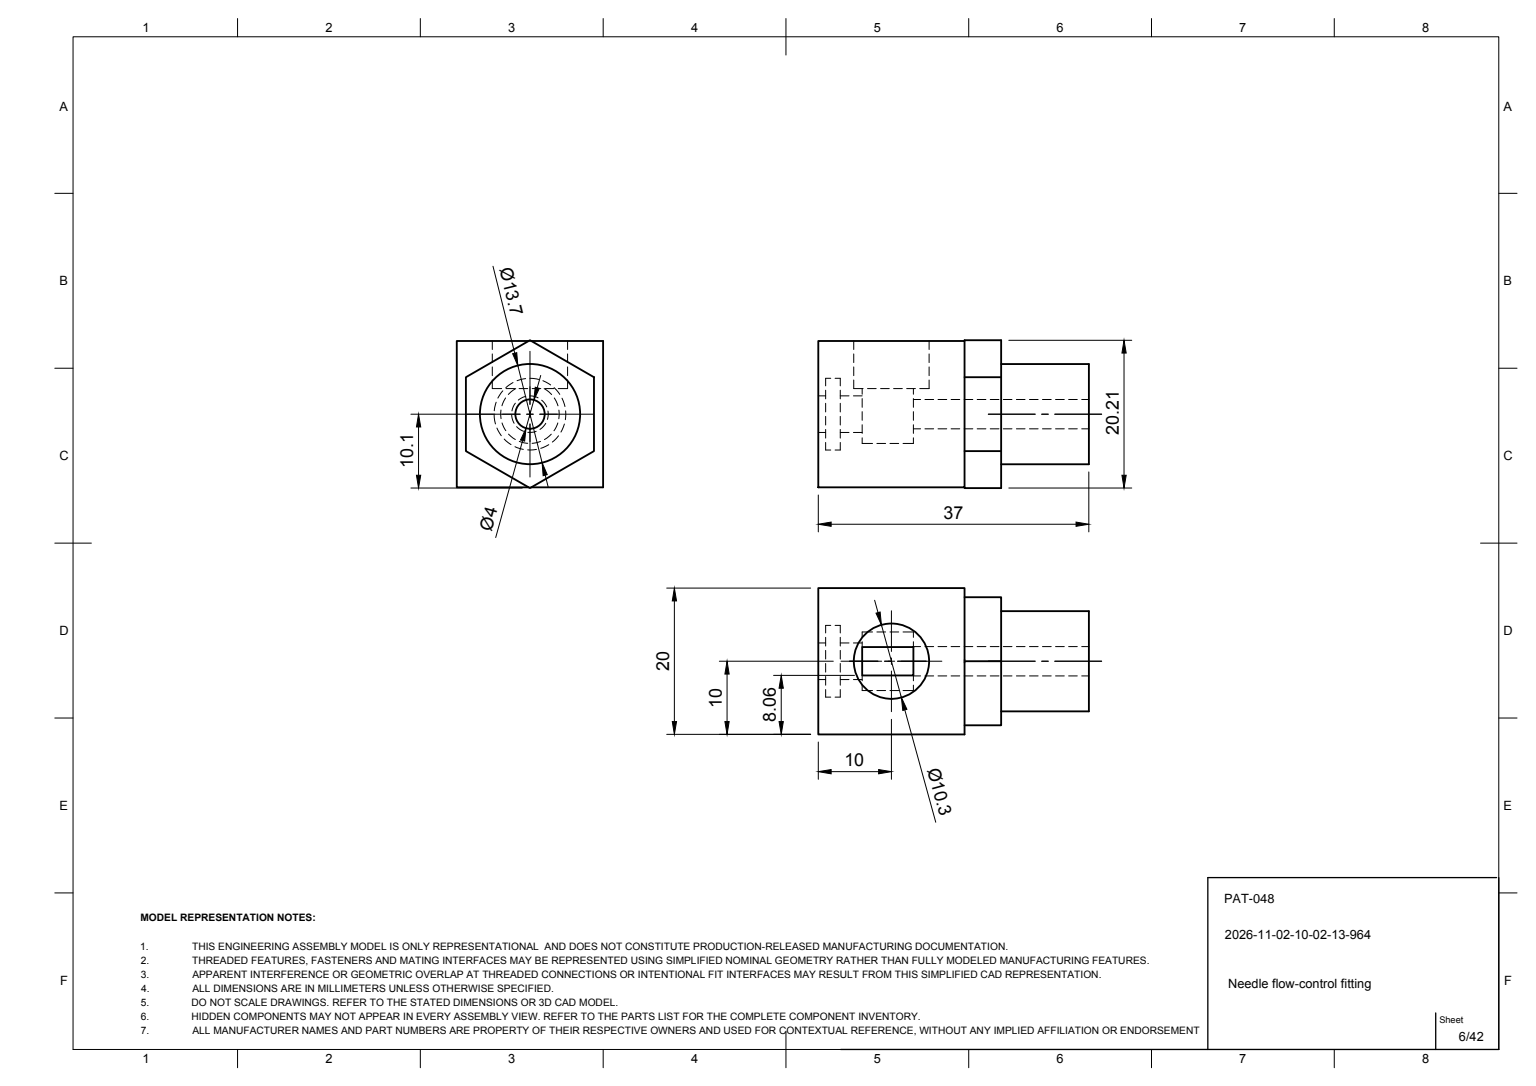
ISO-10303-21;
HEADER;
/* Generated by software containing ST-Developer
 * from STEP Tools, Inc. (www.steptools.com) 
 */

FILE_DESCRIPTION(
/* description */ ('Guided pneumatic stop gate'),
/* implementation_level */ '2;1');

FILE_NAME(
/* name */ 'Needle flow-control fitting.step',
/* time_stamp */ '2026-10-27T21:43:45-07:00',
/* author */ (''),
/* organization */ (''),
/* preprocessor_version */ 'ST-DEVELOPER v20.2',
/* originating_system */ 'Autodesk Translation Framework v15.17.0.0',
/* authorisation */ '');

FILE_SCHEMA (('AUTOMOTIVE_DESIGN { 1 0 10303 214 3 1 1 }'));
ENDSEC;

DATA;
#10=MECHANICAL_DESIGN_GEOMETRIC_PRESENTATION_REPRESENTATION('',(#536),#14392);
#452=SHAPE_REPRESENTATION_RELATIONSHIP('SRR','None',#14586,#494);
#494=ADVANCED_BREP_SHAPE_REPRESENTATION('',(#578),#14348);
#536=STYLED_ITEM('',(#14884),#578);
#578=MANIFOLD_SOLID_BREP('Body1',#7876);
#630=FACE_BOUND('',#1642,.T.);
#631=FACE_BOUND('',#1644,.T.);
#632=FACE_BOUND('',#1648,.T.);
#633=FACE_BOUND('',#1650,.T.);
#634=FACE_BOUND('',#1654,.T.);
#635=FACE_BOUND('',#1658,.T.);
#636=FACE_BOUND('',#1662,.T.);
#637=FACE_BOUND('',#1666,.T.);
#638=FACE_BOUND('',#1677,.T.);
#856=PLANE('',#8460);
#857=PLANE('',#8461);
#858=PLANE('',#8469);
#859=PLANE('',#8471);
#860=PLANE('',#8476);
#861=PLANE('',#8478);
#862=PLANE('',#8479);
#863=PLANE('',#8480);
#864=PLANE('',#8481);
#865=PLANE('',#8482);
#866=PLANE('',#8483);
#867=PLANE('',#8484);
#868=PLANE('',#8485);
#869=PLANE('',#8486);
#870=PLANE('',#8488);
#871=PLANE('',#8489);
#872=PLANE('',#8490);
#873=PLANE('',#8491);
#874=PLANE('',#8492);
#875=PLANE('',#8493);
#876=PLANE('',#8494);
#877=PLANE('',#8499);
#1150=FACE_OUTER_BOUND('',#1640,.T.);
#1151=FACE_OUTER_BOUND('',#1641,.T.);
#1152=FACE_OUTER_BOUND('',#1643,.T.);
#1153=FACE_OUTER_BOUND('',#1645,.T.);
#1154=FACE_OUTER_BOUND('',#1646,.T.);
#1155=FACE_OUTER_BOUND('',#1647,.T.);
#1156=FACE_OUTER_BOUND('',#1649,.T.);
#1157=FACE_OUTER_BOUND('',#1651,.T.);
#1158=FACE_OUTER_BOUND('',#1652,.T.);
#1159=FACE_OUTER_BOUND('',#1653,.T.);
#1160=FACE_OUTER_BOUND('',#1655,.T.);
#1161=FACE_OUTER_BOUND('',#1656,.T.);
#1162=FACE_OUTER_BOUND('',#1657,.T.);
#1163=FACE_OUTER_BOUND('',#1659,.T.);
#1164=FACE_OUTER_BOUND('',#1660,.T.);
#1165=FACE_OUTER_BOUND('',#1661,.T.);
#1166=FACE_OUTER_BOUND('',#1663,.T.);
#1167=FACE_OUTER_BOUND('',#1664,.T.);
#1168=FACE_OUTER_BOUND('',#1665,.T.);
#1169=FACE_OUTER_BOUND('',#1667,.T.);
#1170=FACE_OUTER_BOUND('',#1668,.T.);
#1171=FACE_OUTER_BOUND('',#1669,.T.);
#1172=FACE_OUTER_BOUND('',#1670,.T.);
#1173=FACE_OUTER_BOUND('',#1671,.T.);
#1174=FACE_OUTER_BOUND('',#1672,.T.);
#1175=FACE_OUTER_BOUND('',#1673,.T.);
#1176=FACE_OUTER_BOUND('',#1674,.T.);
#1177=FACE_OUTER_BOUND('',#1675,.T.);
#1178=FACE_OUTER_BOUND('',#1676,.T.);
#1640=EDGE_LOOP('',(#5450,#5451,#5452,#5453));
#1641=EDGE_LOOP('',(#5454));
#1642=EDGE_LOOP('',(#5455,#5456,#5457,#5458));
#1643=EDGE_LOOP('',(#5459,#5460));
#1644=EDGE_LOOP('',(#5461));
#1645=EDGE_LOOP('',(#5462,#5463,#5464,#5465));
#1646=EDGE_LOOP('',(#5466,#5467,#5468,#5469));
#1647=EDGE_LOOP('',(#5470));
#1648=EDGE_LOOP('',(#5471));
#1649=EDGE_LOOP('',(#5472));
#1650=EDGE_LOOP('',(#5473));
#1651=EDGE_LOOP('',(#5474,#5475,#5476,#5477));
#1652=EDGE_LOOP('',(#5478,#5479,#5480,#5481));
#1653=EDGE_LOOP('',(#5482,#5483));
#1654=EDGE_LOOP('',(#5484));
#1655=EDGE_LOOP('',(#5485,#5486,#5487,#5488,#5489,#5490));
#1656=EDGE_LOOP('',(#5491,#5492,#5493,#5494));
#1657=EDGE_LOOP('',(#5495,#5496,#5497,#5498,#5499,#5500));
#1658=EDGE_LOOP('',(#5501));
#1659=EDGE_LOOP('',(#5502,#5503,#5504,#5505));
#1660=EDGE_LOOP('',(#5506,#5507,#5508,#5509,#5510,#5511));
#1661=EDGE_LOOP('',(#5512,#5513,#5514,#5515));
#1662=EDGE_LOOP('',(#5516));
#1663=EDGE_LOOP('',(#5517,#5518,#5519,#5520,#5521,#5522));
#1664=EDGE_LOOP('',(#5523,#5524,#5525));
#1665=EDGE_LOOP('',(#5526,#5527,#5528,#5529,#5530,#5531));
#1666=EDGE_LOOP('',(#5532));
#1667=EDGE_LOOP('',(#5533,#5534,#5535,#5536));
#1668=EDGE_LOOP('',(#5537,#5538,#5539,#5540,#5541));
#1669=EDGE_LOOP('',(#5542,#5543,#5544,#5545,#5546));
#1670=EDGE_LOOP('',(#5547,#5548,#5549,#5550));
#1671=EDGE_LOOP('',(#5551,#5552,#5553,#5554,#5555));
#1672=EDGE_LOOP('',(#5556,#5557,#5558,#5559,#5560));
#1673=EDGE_LOOP('',(#5561,#5562,#5563));
#1674=EDGE_LOOP('',(#5564,#5565,#5566,#5567));
#1675=EDGE_LOOP('',(#5568,#5569,#5570,#5571));
#1676=EDGE_LOOP('',(#5572));
#1677=EDGE_LOOP('',(#5573));
#2308=LINE('',#12067,#2853);
#2309=LINE('',#12072,#2854);
#2310=LINE('',#12074,#2855);
#2311=LINE('',#12076,#2856);
#2312=LINE('',#12077,#2857);
#2313=LINE('',#12088,#2858);
#2314=LINE('',#12097,#2859);
#2315=LINE('',#12100,#2860);
#2316=LINE('',#12108,#2861);
#2317=LINE('',#12110,#2862);
#2318=LINE('',#12112,#2863);
#2319=LINE('',#12114,#2864);
#2320=LINE('',#12116,#2865);
#2321=LINE('',#12117,#2866);
#2322=LINE('',#12121,#2867);
#2323=LINE('',#12123,#2868);
#2324=LINE('',#12125,#2869);
#2325=LINE('',#12126,#2870);
#2326=LINE('',#12129,#2871);
#2327=LINE('',#12130,#2872);
#2328=LINE('',#12132,#2873);
#2329=LINE('',#12133,#2874);
#2330=LINE('',#12136,#2875);
#2331=LINE('',#12137,#2876);
#2332=LINE('',#12140,#2877);
#2333=LINE('',#12141,#2878);
#2334=LINE('',#12142,#2879);
#2335=LINE('',#12146,#2880);
#2336=LINE('',#12148,#2881);
#2337=LINE('',#12149,#2882);
#2338=LINE('',#12152,#2883);
#2339=LINE('',#12153,#2884);
#2340=LINE('',#12157,#2885);
#2341=LINE('',#12159,#2886);
#2342=LINE('',#12161,#2887);
#2343=LINE('',#12163,#2888);
#2344=LINE('',#12165,#2889);
#2345=LINE('',#12166,#2890);
#2346=LINE('',#12170,#2891);
#2347=LINE('',#12171,#2892);
#2348=LINE('',#12174,#2893);
#2349=LINE('',#12175,#2894);
#2350=LINE('',#12177,#2895);
#2351=LINE('',#12178,#2896);
#2352=LINE('',#12180,#2897);
#2353=LINE('',#12182,#2898);
#2354=LINE('',#12187,#2899);
#2355=LINE('',#12191,#2900);
#2853=VECTOR('',#9561,0.515);
#2854=VECTOR('',#9566,1.);
#2855=VECTOR('',#9567,1.);
#2856=VECTOR('',#9568,1.);
#2857=VECTOR('',#9569,1.);
#2858=VECTOR('',#9584,0.49);
#2859=VECTOR('',#9597,0.25);
#2860=VECTOR('',#9600,0.25);
#2861=VECTOR('',#9609,1.);
#2862=VECTOR('',#9610,1.);
#2863=VECTOR('',#9611,1.);
#2864=VECTOR('',#9612,1.);
#2865=VECTOR('',#9613,1.);
#2866=VECTOR('',#9614,1.);
#2867=VECTOR('',#9617,1.);
#2868=VECTOR('',#9618,1.);
#2869=VECTOR('',#9619,1.);
#2870=VECTOR('',#9620,1.);
#2871=VECTOR('',#9623,1.);
#2872=VECTOR('',#9624,1.);
#2873=VECTOR('',#9625,1.);
#2874=VECTOR('',#9626,1.);
#2875=VECTOR('',#9629,1.);
#2876=VECTOR('',#9630,1.);
#2877=VECTOR('',#9633,1.);
#2878=VECTOR('',#9634,1.);
#2879=VECTOR('',#9635,1.);
#2880=VECTOR('',#9640,1.);
#2881=VECTOR('',#9641,1.);
#2882=VECTOR('',#9642,1.);
#2883=VECTOR('',#9645,1.);
#2884=VECTOR('',#9646,1.);
#2885=VECTOR('',#9649,1.);
#2886=VECTOR('',#9650,1.);
#2887=VECTOR('',#9651,1.);
#2888=VECTOR('',#9652,1.);
#2889=VECTOR('',#9653,1.);
#2890=VECTOR('',#9654,1.);
#2891=VECTOR('',#9659,1.);
#2892=VECTOR('',#9660,1.);
#2893=VECTOR('',#9663,1.);
#2894=VECTOR('',#9664,1.);
#2895=VECTOR('',#9667,1.);
#2896=VECTOR('',#9668,1.);
#2897=VECTOR('',#9671,1.);
#2898=VECTOR('',#9674,1.);
#2899=VECTOR('',#9681,0.2);
#2900=VECTOR('',#9686,0.685);
#3398=CIRCLE('',#8458,0.515);
#3399=CIRCLE('',#8459,0.515);
#3400=CIRCLE('',#8462,0.4);
#3401=CIRCLE('',#8463,0.25);
#3402=CIRCLE('',#8465,0.4);
#3403=CIRCLE('',#8467,0.49);
#3404=CIRCLE('',#8468,0.49);
#3405=CIRCLE('',#8470,0.25);
#3406=CIRCLE('',#8472,0.25);
#3407=CIRCLE('',#8475,0.25);
#3408=CIRCLE('',#8477,0.2);
#3409=CIRCLE('',#8487,0.685);
#3410=CIRCLE('',#8496,0.2);
#3411=CIRCLE('',#8498,0.685);
#3777=VERTEX_POINT('',#12064);
#3778=VERTEX_POINT('',#12066);
#3779=VERTEX_POINT('',#12070);
#3780=VERTEX_POINT('',#12071);
#3781=VERTEX_POINT('',#12073);
#3782=VERTEX_POINT('',#12075);
#3783=VERTEX_POINT('',#12080);
#3784=VERTEX_POINT('',#12085);
#3785=VERTEX_POINT('',#12087);
#3786=VERTEX_POINT('',#12091);
#3787=VERTEX_POINT('',#12094);
#3788=VERTEX_POINT('',#12099);
#3789=VERTEX_POINT('',#12103);
#3790=VERTEX_POINT('',#12106);
#3791=VERTEX_POINT('',#12107);
#3792=VERTEX_POINT('',#12109);
#3793=VERTEX_POINT('',#12111);
#3794=VERTEX_POINT('',#12113);
#3795=VERTEX_POINT('',#12115);
#3796=VERTEX_POINT('',#12119);
#3797=VERTEX_POINT('',#12120);
#3798=VERTEX_POINT('',#12122);
#3799=VERTEX_POINT('',#12124);
#3800=VERTEX_POINT('',#12128);
#3801=VERTEX_POINT('',#12131);
#3802=VERTEX_POINT('',#12135);
#3803=VERTEX_POINT('',#12139);
#3804=VERTEX_POINT('',#12145);
#3805=VERTEX_POINT('',#12147);
#3806=VERTEX_POINT('',#12151);
#3807=VERTEX_POINT('',#12155);
#3808=VERTEX_POINT('',#12156);
#3809=VERTEX_POINT('',#12158);
#3810=VERTEX_POINT('',#12160);
#3811=VERTEX_POINT('',#12162);
#3812=VERTEX_POINT('',#12164);
#3813=VERTEX_POINT('',#12167);
#3814=VERTEX_POINT('',#12173);
#3815=VERTEX_POINT('',#12186);
#3816=VERTEX_POINT('',#12190);
#4423=EDGE_CURVE('',#3777,#3777,#3398,.T.);
#4424=EDGE_CURVE('',#3777,#3778,#2308,.T.);
#4425=EDGE_CURVE('',#3778,#3778,#3399,.T.);
#4426=EDGE_CURVE('',#3779,#3780,#2309,.T.);
#4427=EDGE_CURVE('',#3781,#3779,#2310,.T.);
#4428=EDGE_CURVE('',#3782,#3781,#2311,.T.);
#4429=EDGE_CURVE('',#3780,#3782,#2312,.T.);
#4430=EDGE_CURVE('',#3781,#3779,#3400,.T.);
#4431=EDGE_CURVE('',#3783,#3783,#3401,.T.);
#4432=EDGE_CURVE('',#3782,#3780,#3402,.T.);
#4433=EDGE_CURVE('',#3784,#3784,#3403,.T.);
#4434=EDGE_CURVE('',#3784,#3785,#2313,.T.);
#4435=EDGE_CURVE('',#3785,#3785,#3404,.T.);
#4436=EDGE_CURVE('',#3786,#3786,#3405,.T.);
#4437=EDGE_CURVE('',#3787,#3787,#3406,.T.);
#4438=EDGE_CURVE('',#3783,#3787,#2314,.T.);
#4439=EDGE_CURVE('',#3786,#3788,#2315,.T.);
#4440=EDGE_CURVE('',#3788,#3788,#3407,.T.);
#4441=EDGE_CURVE('',#3789,#3789,#3408,.T.);
#4442=EDGE_CURVE('',#3790,#3791,#2316,.T.);
#4443=EDGE_CURVE('',#3791,#3792,#2317,.T.);
#4444=EDGE_CURVE('',#3792,#3793,#2318,.T.);
#4445=EDGE_CURVE('',#3794,#3793,#2319,.T.);
#4446=EDGE_CURVE('',#3795,#3794,#2320,.T.);
#4447=EDGE_CURVE('',#3790,#3795,#2321,.T.);
#4448=EDGE_CURVE('',#3796,#3797,#2322,.T.);
#4449=EDGE_CURVE('',#3797,#3798,#2323,.T.);
#4450=EDGE_CURVE('',#3799,#3798,#2324,.T.);
#4451=EDGE_CURVE('',#3796,#3799,#2325,.T.);
#4452=EDGE_CURVE('',#3800,#3793,#2326,.T.);
#4453=EDGE_CURVE('',#3800,#3796,#2327,.T.);
#4454=EDGE_CURVE('',#3801,#3799,#2328,.T.);
#4455=EDGE_CURVE('',#3794,#3801,#2329,.T.);
#4456=EDGE_CURVE('',#3802,#3801,#2330,.T.);
#4457=EDGE_CURVE('',#3795,#3802,#2331,.T.);
#4458=EDGE_CURVE('',#3797,#3803,#2332,.T.);
#4459=EDGE_CURVE('',#3790,#3803,#2333,.T.);
#4460=EDGE_CURVE('',#3798,#3802,#2334,.T.);
#4461=EDGE_CURVE('',#3804,#3803,#2335,.T.);
#4462=EDGE_CURVE('',#3800,#3805,#2336,.T.);
#4463=EDGE_CURVE('',#3805,#3804,#2337,.T.);
#4464=EDGE_CURVE('',#3793,#3806,#2338,.T.);
#4465=EDGE_CURVE('',#3806,#3800,#2339,.T.);
#4466=EDGE_CURVE('',#3807,#3808,#2340,.T.);
#4467=EDGE_CURVE('',#3809,#3807,#2341,.T.);
#4468=EDGE_CURVE('',#3810,#3809,#2342,.T.);
#4469=EDGE_CURVE('',#3811,#3810,#2343,.T.);
#4470=EDGE_CURVE('',#3812,#3811,#2344,.T.);
#4471=EDGE_CURVE('',#3808,#3812,#2345,.T.);
#4472=EDGE_CURVE('',#3813,#3813,#3409,.T.);
#4473=EDGE_CURVE('',#3807,#3792,#2346,.T.);
#4474=EDGE_CURVE('',#3809,#3791,#2347,.T.);
#4475=EDGE_CURVE('',#3814,#3790,#2348,.T.);
#4476=EDGE_CURVE('',#3810,#3814,#2349,.T.);
#4477=EDGE_CURVE('',#3803,#3814,#2350,.T.);
#4478=EDGE_CURVE('',#3811,#3804,#2351,.T.);
#4479=EDGE_CURVE('',#3812,#3805,#2352,.T.);
#4480=EDGE_CURVE('',#3808,#3806,#2353,.T.);
#4481=EDGE_CURVE('',#3789,#3815,#2354,.T.);
#4482=EDGE_CURVE('',#3815,#3815,#3410,.T.);
#4483=EDGE_CURVE('',#3813,#3816,#2355,.T.);
#4484=EDGE_CURVE('',#3816,#3816,#3411,.T.);
#5450=ORIENTED_EDGE('',*,*,#4423,.F.);
#5451=ORIENTED_EDGE('',*,*,#4424,.T.);
#5452=ORIENTED_EDGE('',*,*,#4425,.F.);
#5453=ORIENTED_EDGE('',*,*,#4424,.F.);
#5454=ORIENTED_EDGE('',*,*,#4423,.T.);
#5455=ORIENTED_EDGE('',*,*,#4426,.F.);
#5456=ORIENTED_EDGE('',*,*,#4427,.F.);
#5457=ORIENTED_EDGE('',*,*,#4428,.F.);
#5458=ORIENTED_EDGE('',*,*,#4429,.F.);
#5459=ORIENTED_EDGE('',*,*,#4427,.T.);
#5460=ORIENTED_EDGE('',*,*,#4430,.F.);
#5461=ORIENTED_EDGE('',*,*,#4431,.T.);
#5462=ORIENTED_EDGE('',*,*,#4428,.T.);
#5463=ORIENTED_EDGE('',*,*,#4430,.T.);
#5464=ORIENTED_EDGE('',*,*,#4426,.T.);
#5465=ORIENTED_EDGE('',*,*,#4432,.F.);
#5466=ORIENTED_EDGE('',*,*,#4433,.F.);
#5467=ORIENTED_EDGE('',*,*,#4434,.T.);
#5468=ORIENTED_EDGE('',*,*,#4435,.T.);
#5469=ORIENTED_EDGE('',*,*,#4434,.F.);
#5470=ORIENTED_EDGE('',*,*,#4435,.F.);
#5471=ORIENTED_EDGE('',*,*,#4436,.F.);
#5472=ORIENTED_EDGE('',*,*,#4433,.T.);
#5473=ORIENTED_EDGE('',*,*,#4437,.F.);
#5474=ORIENTED_EDGE('',*,*,#4431,.F.);
#5475=ORIENTED_EDGE('',*,*,#4438,.T.);
#5476=ORIENTED_EDGE('',*,*,#4437,.T.);
#5477=ORIENTED_EDGE('',*,*,#4438,.F.);
#5478=ORIENTED_EDGE('',*,*,#4436,.T.);
#5479=ORIENTED_EDGE('',*,*,#4439,.T.);
#5480=ORIENTED_EDGE('',*,*,#4440,.F.);
#5481=ORIENTED_EDGE('',*,*,#4439,.F.);
#5482=ORIENTED_EDGE('',*,*,#4429,.T.);
#5483=ORIENTED_EDGE('',*,*,#4432,.T.);
#5484=ORIENTED_EDGE('',*,*,#4441,.F.);
#5485=ORIENTED_EDGE('',*,*,#4442,.T.);
#5486=ORIENTED_EDGE('',*,*,#4443,.T.);
#5487=ORIENTED_EDGE('',*,*,#4444,.T.);
#5488=ORIENTED_EDGE('',*,*,#4445,.F.);
#5489=ORIENTED_EDGE('',*,*,#4446,.F.);
#5490=ORIENTED_EDGE('',*,*,#4447,.F.);
#5491=ORIENTED_EDGE('',*,*,#4448,.T.);
#5492=ORIENTED_EDGE('',*,*,#4449,.T.);
#5493=ORIENTED_EDGE('',*,*,#4450,.F.);
#5494=ORIENTED_EDGE('',*,*,#4451,.F.);
#5495=ORIENTED_EDGE('',*,*,#4445,.T.);
#5496=ORIENTED_EDGE('',*,*,#4452,.F.);
#5497=ORIENTED_EDGE('',*,*,#4453,.T.);
#5498=ORIENTED_EDGE('',*,*,#4451,.T.);
#5499=ORIENTED_EDGE('',*,*,#4454,.F.);
#5500=ORIENTED_EDGE('',*,*,#4455,.F.);
#5501=ORIENTED_EDGE('',*,*,#4425,.T.);
#5502=ORIENTED_EDGE('',*,*,#4446,.T.);
#5503=ORIENTED_EDGE('',*,*,#4455,.T.);
#5504=ORIENTED_EDGE('',*,*,#4456,.F.);
#5505=ORIENTED_EDGE('',*,*,#4457,.F.);
#5506=ORIENTED_EDGE('',*,*,#4458,.T.);
#5507=ORIENTED_EDGE('',*,*,#4459,.F.);
#5508=ORIENTED_EDGE('',*,*,#4447,.T.);
#5509=ORIENTED_EDGE('',*,*,#4457,.T.);
#5510=ORIENTED_EDGE('',*,*,#4460,.F.);
#5511=ORIENTED_EDGE('',*,*,#4449,.F.);
#5512=ORIENTED_EDGE('',*,*,#4460,.T.);
#5513=ORIENTED_EDGE('',*,*,#4456,.T.);
#5514=ORIENTED_EDGE('',*,*,#4454,.T.);
#5515=ORIENTED_EDGE('',*,*,#4450,.T.);
#5516=ORIENTED_EDGE('',*,*,#4440,.T.);
#5517=ORIENTED_EDGE('',*,*,#4461,.T.);
#5518=ORIENTED_EDGE('',*,*,#4458,.F.);
#5519=ORIENTED_EDGE('',*,*,#4448,.F.);
#5520=ORIENTED_EDGE('',*,*,#4453,.F.);
#5521=ORIENTED_EDGE('',*,*,#4462,.T.);
#5522=ORIENTED_EDGE('',*,*,#4463,.T.);
#5523=ORIENTED_EDGE('',*,*,#4452,.T.);
#5524=ORIENTED_EDGE('',*,*,#4464,.T.);
#5525=ORIENTED_EDGE('',*,*,#4465,.T.);
#5526=ORIENTED_EDGE('',*,*,#4466,.F.);
#5527=ORIENTED_EDGE('',*,*,#4467,.F.);
#5528=ORIENTED_EDGE('',*,*,#4468,.F.);
#5529=ORIENTED_EDGE('',*,*,#4469,.F.);
#5530=ORIENTED_EDGE('',*,*,#4470,.F.);
#5531=ORIENTED_EDGE('',*,*,#4471,.F.);
#5532=ORIENTED_EDGE('',*,*,#4472,.T.);
#5533=ORIENTED_EDGE('',*,*,#4467,.T.);
#5534=ORIENTED_EDGE('',*,*,#4473,.T.);
#5535=ORIENTED_EDGE('',*,*,#4443,.F.);
#5536=ORIENTED_EDGE('',*,*,#4474,.F.);
#5537=ORIENTED_EDGE('',*,*,#4468,.T.);
#5538=ORIENTED_EDGE('',*,*,#4474,.T.);
#5539=ORIENTED_EDGE('',*,*,#4442,.F.);
#5540=ORIENTED_EDGE('',*,*,#4475,.F.);
#5541=ORIENTED_EDGE('',*,*,#4476,.F.);
#5542=ORIENTED_EDGE('',*,*,#4469,.T.);
#5543=ORIENTED_EDGE('',*,*,#4476,.T.);
#5544=ORIENTED_EDGE('',*,*,#4477,.F.);
#5545=ORIENTED_EDGE('',*,*,#4461,.F.);
#5546=ORIENTED_EDGE('',*,*,#4478,.F.);
#5547=ORIENTED_EDGE('',*,*,#4470,.T.);
#5548=ORIENTED_EDGE('',*,*,#4478,.T.);
#5549=ORIENTED_EDGE('',*,*,#4463,.F.);
#5550=ORIENTED_EDGE('',*,*,#4479,.F.);
#5551=ORIENTED_EDGE('',*,*,#4471,.T.);
#5552=ORIENTED_EDGE('',*,*,#4479,.T.);
#5553=ORIENTED_EDGE('',*,*,#4462,.F.);
#5554=ORIENTED_EDGE('',*,*,#4465,.F.);
#5555=ORIENTED_EDGE('',*,*,#4480,.F.);
#5556=ORIENTED_EDGE('',*,*,#4466,.T.);
#5557=ORIENTED_EDGE('',*,*,#4480,.T.);
#5558=ORIENTED_EDGE('',*,*,#4464,.F.);
#5559=ORIENTED_EDGE('',*,*,#4444,.F.);
#5560=ORIENTED_EDGE('',*,*,#4473,.F.);
#5561=ORIENTED_EDGE('',*,*,#4459,.T.);
#5562=ORIENTED_EDGE('',*,*,#4477,.T.);
#5563=ORIENTED_EDGE('',*,*,#4475,.T.);
#5564=ORIENTED_EDGE('',*,*,#4441,.T.);
#5565=ORIENTED_EDGE('',*,*,#4481,.T.);
#5566=ORIENTED_EDGE('',*,*,#4482,.T.);
#5567=ORIENTED_EDGE('',*,*,#4481,.F.);
#5568=ORIENTED_EDGE('',*,*,#4472,.F.);
#5569=ORIENTED_EDGE('',*,*,#4483,.T.);
#5570=ORIENTED_EDGE('',*,*,#4484,.T.);
#5571=ORIENTED_EDGE('',*,*,#4483,.F.);
#5572=ORIENTED_EDGE('',*,*,#4484,.F.);
#5573=ORIENTED_EDGE('',*,*,#4482,.F.);
#7251=CYLINDRICAL_SURFACE('',#8457,0.515);
#7252=CYLINDRICAL_SURFACE('',#8464,0.4);
#7253=CYLINDRICAL_SURFACE('',#8466,0.49);
#7254=CYLINDRICAL_SURFACE('',#8473,0.25);
#7255=CYLINDRICAL_SURFACE('',#8474,0.25);
#7256=CYLINDRICAL_SURFACE('',#8495,0.2);
#7257=CYLINDRICAL_SURFACE('',#8497,0.685);
#7432=ADVANCED_FACE('',(#1150),#7251,.F.);
#7433=ADVANCED_FACE('',(#1151,#630),#856,.T.);
#7434=ADVANCED_FACE('',(#1152,#631),#857,.F.);
#7435=ADVANCED_FACE('',(#1153),#7252,.F.);
#7436=ADVANCED_FACE('',(#1154),#7253,.F.);
#7437=ADVANCED_FACE('',(#1155,#632),#858,.F.);
#7438=ADVANCED_FACE('',(#1156,#633),#859,.T.);
#7439=ADVANCED_FACE('',(#1157),#7254,.F.);
#7440=ADVANCED_FACE('',(#1158),#7255,.F.);
#7441=ADVANCED_FACE('',(#1159,#634),#860,.T.);
#7442=ADVANCED_FACE('',(#1160),#861,.F.);
#7443=ADVANCED_FACE('',(#1161),#862,.T.);
#7444=ADVANCED_FACE('',(#1162,#635),#863,.T.);
#7445=ADVANCED_FACE('',(#1163),#864,.T.);
#7446=ADVANCED_FACE('',(#1164),#865,.T.);
#7447=ADVANCED_FACE('',(#1165,#636),#866,.T.);
#7448=ADVANCED_FACE('',(#1166),#867,.F.);
#7449=ADVANCED_FACE('',(#1167),#868,.T.);
#7450=ADVANCED_FACE('',(#1168,#637),#869,.F.);
#7451=ADVANCED_FACE('',(#1169),#870,.T.);
#7452=ADVANCED_FACE('',(#1170),#871,.T.);
#7453=ADVANCED_FACE('',(#1171),#872,.T.);
#7454=ADVANCED_FACE('',(#1172),#873,.T.);
#7455=ADVANCED_FACE('',(#1173),#874,.T.);
#7456=ADVANCED_FACE('',(#1174),#875,.T.);
#7457=ADVANCED_FACE('',(#1175),#876,.T.);
#7458=ADVANCED_FACE('',(#1176),#7256,.F.);
#7459=ADVANCED_FACE('',(#1177),#7257,.T.);
#7460=ADVANCED_FACE('',(#1178,#638),#877,.F.);
#7876=CLOSED_SHELL('',(#7432,#7433,#7434,#7435,#7436,#7437,#7438,#7439,
#7440,#7441,#7442,#7443,#7444,#7445,#7446,#7447,#7448,#7449,#7450,#7451,
#7452,#7453,#7454,#7455,#7456,#7457,#7458,#7459,#7460));
#8456=AXIS2_PLACEMENT_3D('',#12062,#9555,#9556);
#8457=AXIS2_PLACEMENT_3D('',#12063,#9557,#9558);
#8458=AXIS2_PLACEMENT_3D('',#12065,#9559,#9560);
#8459=AXIS2_PLACEMENT_3D('',#12068,#9562,#9563);
#8460=AXIS2_PLACEMENT_3D('',#12069,#9564,#9565);
#8461=AXIS2_PLACEMENT_3D('',#12078,#9570,#9571);
#8462=AXIS2_PLACEMENT_3D('',#12079,#9572,#9573);
#8463=AXIS2_PLACEMENT_3D('',#12081,#9574,#9575);
#8464=AXIS2_PLACEMENT_3D('',#12082,#9576,#9577);
#8465=AXIS2_PLACEMENT_3D('',#12083,#9578,#9579);
#8466=AXIS2_PLACEMENT_3D('',#12084,#9580,#9581);
#8467=AXIS2_PLACEMENT_3D('',#12086,#9582,#9583);
#8468=AXIS2_PLACEMENT_3D('',#12089,#9585,#9586);
#8469=AXIS2_PLACEMENT_3D('',#12090,#9587,#9588);
#8470=AXIS2_PLACEMENT_3D('',#12092,#9589,#9590);
#8471=AXIS2_PLACEMENT_3D('',#12093,#9591,#9592);
#8472=AXIS2_PLACEMENT_3D('',#12095,#9593,#9594);
#8473=AXIS2_PLACEMENT_3D('',#12096,#9595,#9596);
#8474=AXIS2_PLACEMENT_3D('',#12098,#9598,#9599);
#8475=AXIS2_PLACEMENT_3D('',#12101,#9601,#9602);
#8476=AXIS2_PLACEMENT_3D('',#12102,#9603,#9604);
#8477=AXIS2_PLACEMENT_3D('',#12104,#9605,#9606);
#8478=AXIS2_PLACEMENT_3D('',#12105,#9607,#9608);
#8479=AXIS2_PLACEMENT_3D('',#12118,#9615,#9616);
#8480=AXIS2_PLACEMENT_3D('',#12127,#9621,#9622);
#8481=AXIS2_PLACEMENT_3D('',#12134,#9627,#9628);
#8482=AXIS2_PLACEMENT_3D('',#12138,#9631,#9632);
#8483=AXIS2_PLACEMENT_3D('',#12143,#9636,#9637);
#8484=AXIS2_PLACEMENT_3D('',#12144,#9638,#9639);
#8485=AXIS2_PLACEMENT_3D('',#12150,#9643,#9644);
#8486=AXIS2_PLACEMENT_3D('',#12154,#9647,#9648);
#8487=AXIS2_PLACEMENT_3D('',#12168,#9655,#9656);
#8488=AXIS2_PLACEMENT_3D('',#12169,#9657,#9658);
#8489=AXIS2_PLACEMENT_3D('',#12172,#9661,#9662);
#8490=AXIS2_PLACEMENT_3D('',#12176,#9665,#9666);
#8491=AXIS2_PLACEMENT_3D('',#12179,#9669,#9670);
#8492=AXIS2_PLACEMENT_3D('',#12181,#9672,#9673);
#8493=AXIS2_PLACEMENT_3D('',#12183,#9675,#9676);
#8494=AXIS2_PLACEMENT_3D('',#12184,#9677,#9678);
#8495=AXIS2_PLACEMENT_3D('',#12185,#9679,#9680);
#8496=AXIS2_PLACEMENT_3D('',#12188,#9682,#9683);
#8497=AXIS2_PLACEMENT_3D('',#12189,#9684,#9685);
#8498=AXIS2_PLACEMENT_3D('',#12192,#9687,#9688);
#8499=AXIS2_PLACEMENT_3D('',#12193,#9689,#9690);
#9555=DIRECTION('axis',(0.,0.,1.));
#9556=DIRECTION('refdir',(1.,0.,0.));
#9557=DIRECTION('center_axis',(1.,0.,0.));
#9558=DIRECTION('ref_axis',(0.,0.,-1.));
#9559=DIRECTION('center_axis',(1.,0.,0.));
#9560=DIRECTION('ref_axis',(0.,0.,-1.));
#9561=DIRECTION('',(1.,0.,0.));
#9562=DIRECTION('center_axis',(-1.,0.,0.));
#9563=DIRECTION('ref_axis',(0.,0.,-1.));
#9564=DIRECTION('center_axis',(1.,0.,0.));
#9565=DIRECTION('ref_axis',(0.,0.,-1.));
#9566=DIRECTION('',(0.,0.,-1.));
#9567=DIRECTION('',(0.,-1.,0.));
#9568=DIRECTION('',(0.,0.,1.));
#9569=DIRECTION('',(0.,1.,0.));
#9570=DIRECTION('center_axis',(0.,0.,1.));
#9571=DIRECTION('ref_axis',(1.,0.,0.));
#9572=DIRECTION('center_axis',(0.,0.,1.));
#9573=DIRECTION('ref_axis',(1.,0.,0.));
#9574=DIRECTION('center_axis',(0.,0.,1.));
#9575=DIRECTION('ref_axis',(1.,0.,0.));
#9576=DIRECTION('center_axis',(0.,0.,1.));
#9577=DIRECTION('ref_axis',(-1.,1.22464679914735E-16,0.));
#9578=DIRECTION('center_axis',(0.,0.,1.));
#9579=DIRECTION('ref_axis',(1.,0.,0.));
#9580=DIRECTION('center_axis',(0.,0.,1.));
#9581=DIRECTION('ref_axis',(1.,0.,0.));
#9582=DIRECTION('center_axis',(0.,0.,1.));
#9583=DIRECTION('ref_axis',(1.,0.,0.));
#9584=DIRECTION('',(0.,0.,1.));
#9585=DIRECTION('center_axis',(0.,0.,1.));
#9586=DIRECTION('ref_axis',(1.,0.,0.));
#9587=DIRECTION('center_axis',(0.,0.,1.));
#9588=DIRECTION('ref_axis',(1.,0.,0.));
#9589=DIRECTION('center_axis',(0.,0.,-1.));
#9590=DIRECTION('ref_axis',(1.,0.,0.));
#9591=DIRECTION('center_axis',(0.,0.,1.));
#9592=DIRECTION('ref_axis',(1.,0.,0.));
#9593=DIRECTION('center_axis',(0.,0.,1.));
#9594=DIRECTION('ref_axis',(1.,0.,0.));
#9595=DIRECTION('center_axis',(0.,0.,1.));
#9596=DIRECTION('ref_axis',(1.,0.,0.));
#9597=DIRECTION('',(0.,0.,1.));
#9598=DIRECTION('center_axis',(0.,0.,1.));
#9599=DIRECTION('ref_axis',(1.,0.,0.));
#9600=DIRECTION('',(0.,0.,1.));
#9601=DIRECTION('center_axis',(0.,0.,-1.));
#9602=DIRECTION('ref_axis',(1.,0.,0.));
#9603=DIRECTION('center_axis',(0.,0.,1.));
#9604=DIRECTION('ref_axis',(1.,0.,0.));
#9605=DIRECTION('center_axis',(0.,0.,1.));
#9606=DIRECTION('ref_axis',(1.,0.,0.));
#9607=DIRECTION('center_axis',(0.,0.,1.));
#9608=DIRECTION('ref_axis',(1.,0.,0.));
#9609=DIRECTION('',(0.5,-0.866025403784439,0.));
#9610=DIRECTION('',(1.,-3.43386193997065E-16,0.));
#9611=DIRECTION('',(0.5,0.866025403784439,0.));
#9612=DIRECTION('',(0.,1.,0.));
#9613=DIRECTION('',(1.,0.,0.));
#9614=DIRECTION('',(0.,-1.,0.));
#9615=DIRECTION('center_axis',(0.,1.,0.));
#9616=DIRECTION('ref_axis',(-1.,0.,0.));
#9617=DIRECTION('',(-1.,0.,0.));
#9618=DIRECTION('',(0.,0.,1.));
#9619=DIRECTION('',(-1.,0.,0.));
#9620=DIRECTION('',(0.,0.,1.));
#9621=DIRECTION('center_axis',(1.,0.,0.));
#9622=DIRECTION('ref_axis',(0.,1.,0.));
#9623=DIRECTION('',(0.,-1.,0.));
#9624=DIRECTION('',(0.,1.,0.));
#9625=DIRECTION('',(0.,1.,0.));
#9626=DIRECTION('',(0.,0.,1.));
#9627=DIRECTION('center_axis',(0.,-1.,0.));
#9628=DIRECTION('ref_axis',(1.,0.,0.));
#9629=DIRECTION('',(1.,0.,0.));
#9630=DIRECTION('',(0.,0.,1.));
#9631=DIRECTION('center_axis',(-1.,0.,0.));
#9632=DIRECTION('ref_axis',(0.,-1.,0.));
#9633=DIRECTION('',(0.,-1.,0.));
#9634=DIRECTION('',(0.,1.,0.));
#9635=DIRECTION('',(0.,-1.,0.));
#9636=DIRECTION('center_axis',(0.,0.,1.));
#9637=DIRECTION('ref_axis',(1.,0.,0.));
#9638=DIRECTION('center_axis',(0.,0.,1.));
#9639=DIRECTION('ref_axis',(1.,0.,0.));
#9640=DIRECTION('',(-0.5,-0.866025403784439,0.));
#9641=DIRECTION('',(-0.5,0.866025403784439,0.));
#9642=DIRECTION('',(-1.,0.,0.));
#9643=DIRECTION('center_axis',(0.,0.,1.));
#9644=DIRECTION('ref_axis',(1.,0.,0.));
#9645=DIRECTION('',(0.5,0.866025403784439,0.));
#9646=DIRECTION('',(-0.5,0.866025403784439,0.));
#9647=DIRECTION('center_axis',(0.,0.,1.));
#9648=DIRECTION('ref_axis',(1.,0.,0.));
#9649=DIRECTION('',(0.5,0.866025403784439,0.));
#9650=DIRECTION('',(1.,-3.43386193997065E-16,0.));
#9651=DIRECTION('',(0.5,-0.866025403784439,0.));
#9652=DIRECTION('',(-0.5,-0.866025403784438,0.));
#9653=DIRECTION('',(-1.,0.,0.));
#9654=DIRECTION('',(-0.5,0.866025403784439,0.));
#9655=DIRECTION('center_axis',(0.,0.,1.));
#9656=DIRECTION('ref_axis',(1.,0.,0.));
#9657=DIRECTION('center_axis',(-3.43386193997065E-16,-1.,0.));
#9658=DIRECTION('ref_axis',(1.,-3.43386193997065E-16,0.));
#9659=DIRECTION('',(0.,0.,1.));
#9660=DIRECTION('',(0.,0.,1.));
#9661=DIRECTION('center_axis',(-0.866025403784439,-0.5,0.));
#9662=DIRECTION('ref_axis',(0.5,-0.866025403784439,0.));
#9663=DIRECTION('',(0.5,-0.866025403784439,0.));
#9664=DIRECTION('',(0.,0.,1.));
#9665=DIRECTION('center_axis',(-0.866025403784439,0.5,0.));
#9666=DIRECTION('ref_axis',(-0.5,-0.866025403784439,0.));
#9667=DIRECTION('',(-0.5,-0.866025403784438,0.));
#9668=DIRECTION('',(0.,0.,1.));
#9669=DIRECTION('center_axis',(0.,1.,0.));
#9670=DIRECTION('ref_axis',(-1.,0.,0.));
#9671=DIRECTION('',(0.,0.,1.));
#9672=DIRECTION('center_axis',(0.866025403784439,0.5,0.));
#9673=DIRECTION('ref_axis',(-0.5,0.866025403784439,0.));
#9674=DIRECTION('',(0.,0.,1.));
#9675=DIRECTION('center_axis',(0.866025403784439,-0.5,0.));
#9676=DIRECTION('ref_axis',(0.5,0.866025403784439,0.));
#9677=DIRECTION('center_axis',(0.,0.,1.));
#9678=DIRECTION('ref_axis',(1.,0.,0.));
#9679=DIRECTION('center_axis',(0.,0.,1.));
#9680=DIRECTION('ref_axis',(1.,0.,0.));
#9681=DIRECTION('',(0.,0.,-1.));
#9682=DIRECTION('center_axis',(0.,0.,-1.));
#9683=DIRECTION('ref_axis',(1.,0.,0.));
#9684=DIRECTION('center_axis',(0.,0.,1.));
#9685=DIRECTION('ref_axis',(1.,0.,0.));
#9686=DIRECTION('',(0.,0.,-1.));
#9687=DIRECTION('center_axis',(0.,0.,1.));
#9688=DIRECTION('ref_axis',(1.,0.,0.));
#9689=DIRECTION('center_axis',(0.,0.,1.));
#9690=DIRECTION('ref_axis',(1.,0.,0.));
#12062=CARTESIAN_POINT('',(0.,0.,0.));
#12063=CARTESIAN_POINT('Origin',(0.35,0.8,8.5));
#12064=CARTESIAN_POINT('',(0.35,0.8,9.015));
#12065=CARTESIAN_POINT('Origin',(0.35,0.8,8.5));
#12066=CARTESIAN_POINT('',(1.,0.8,9.015));
#12067=CARTESIAN_POINT('',(0.35,0.8,9.015));
#12068=CARTESIAN_POINT('Origin',(1.,0.8,8.5));
#12069=CARTESIAN_POINT('Origin',(0.35,0.8,8.5));
#12070=CARTESIAN_POINT('',(0.35,0.606350832689629,8.9));
#12071=CARTESIAN_POINT('',(0.35,0.606350832689629,8.2));
#12072=CARTESIAN_POINT('',(0.35,0.606350832689629,8.2));
#12073=CARTESIAN_POINT('',(0.35,0.993649167310371,8.9));
#12074=CARTESIAN_POINT('',(0.35,0.8,8.9));
#12075=CARTESIAN_POINT('',(0.35,0.993649167310371,8.2));
#12076=CARTESIAN_POINT('',(0.35,0.993649167310371,8.2));
#12077=CARTESIAN_POINT('',(0.35,0.8,8.2));
#12078=CARTESIAN_POINT('Origin',(0.,0.8,8.9));
#12079=CARTESIAN_POINT('Origin',(0.,0.8,8.9));
#12080=CARTESIAN_POINT('',(-0.25,0.8,8.9));
#12081=CARTESIAN_POINT('Origin',(0.,0.8,8.9));
#12082=CARTESIAN_POINT('Origin',(0.,0.8,8.2));
#12083=CARTESIAN_POINT('Origin',(0.,0.8,8.2));
#12084=CARTESIAN_POINT('Origin',(0.,0.8,9.2));
#12085=CARTESIAN_POINT('',(-0.49,0.8,9.2));
#12086=CARTESIAN_POINT('Origin',(0.,0.8,9.2));
#12087=CARTESIAN_POINT('',(-0.49,0.8,9.4));
#12088=CARTESIAN_POINT('',(-0.49,0.8,9.2));
#12089=CARTESIAN_POINT('Origin',(0.,0.8,9.4));
#12090=CARTESIAN_POINT('Origin',(0.,0.8,9.4));
#12091=CARTESIAN_POINT('',(-0.25,0.8,9.4));
#12092=CARTESIAN_POINT('Origin',(0.,0.8,9.4));
#12093=CARTESIAN_POINT('Origin',(0.,0.8,9.2));
#12094=CARTESIAN_POINT('',(-0.25,0.8,9.2));
#12095=CARTESIAN_POINT('Origin',(0.,0.8,9.2));
#12096=CARTESIAN_POINT('Origin',(0.,0.8,8.8));
#12097=CARTESIAN_POINT('',(-0.25,0.8,8.8));
#12098=CARTESIAN_POINT('Origin',(0.,0.8,8.8));
#12099=CARTESIAN_POINT('',(-0.25,0.8,9.5));
#12100=CARTESIAN_POINT('',(-0.25,0.8,8.8));
#12101=CARTESIAN_POINT('Origin',(0.,0.8,9.5));
#12102=CARTESIAN_POINT('Origin',(0.,0.8,8.2));
#12103=CARTESIAN_POINT('',(-0.2,0.8,8.2));
#12104=CARTESIAN_POINT('Origin',(0.,0.8,8.2));
#12105=CARTESIAN_POINT('Origin',(0.,0.8,7.5));
#12106=CARTESIAN_POINT('',(-1.,0.782050807568877,7.5));
#12107=CARTESIAN_POINT('',(-0.505181485540923,-0.0749999999999997,7.5));
#12108=CARTESIAN_POINT('',(-1.01036297108185,0.8,7.5));
#12109=CARTESIAN_POINT('',(0.505181485540923,-0.075,7.5));
#12110=CARTESIAN_POINT('',(-0.505181485540923,-0.0749999999999997,7.5));
#12111=CARTESIAN_POINT('',(1.,0.782050807568877,7.5));
#12112=CARTESIAN_POINT('',(0.505181485540923,-0.075,7.5));
#12113=CARTESIAN_POINT('',(1.,-0.2,7.5));
#12114=CARTESIAN_POINT('',(1.,-0.2,7.5));
#12115=CARTESIAN_POINT('',(-1.,-0.2,7.5));
#12116=CARTESIAN_POINT('',(-1.,-0.2,7.5));
#12117=CARTESIAN_POINT('',(-1.,1.8,7.5));
#12118=CARTESIAN_POINT('Origin',(1.,1.8,7.5));
#12119=CARTESIAN_POINT('',(1.,1.8,7.5));
#12120=CARTESIAN_POINT('',(-1.,1.8,7.5));
#12121=CARTESIAN_POINT('',(1.,1.8,7.5));
#12122=CARTESIAN_POINT('',(-1.,1.8,9.5));
#12123=CARTESIAN_POINT('',(-1.,1.8,7.5));
#12124=CARTESIAN_POINT('',(1.,1.8,9.5));
#12125=CARTESIAN_POINT('',(1.,1.8,9.5));
#12126=CARTESIAN_POINT('',(1.,1.8,7.5));
#12127=CARTESIAN_POINT('Origin',(1.,-0.2,7.5));
#12128=CARTESIAN_POINT('',(1.,0.817949192431123,7.5));
#12129=CARTESIAN_POINT('',(1.,0.3,7.5));
#12130=CARTESIAN_POINT('',(1.,-0.2,7.5));
#12131=CARTESIAN_POINT('',(1.,-0.2,9.5));
#12132=CARTESIAN_POINT('',(1.,-0.2,9.5));
#12133=CARTESIAN_POINT('',(1.,-0.2,7.5));
#12134=CARTESIAN_POINT('Origin',(-1.,-0.2,7.5));
#12135=CARTESIAN_POINT('',(-1.,-0.2,9.5));
#12136=CARTESIAN_POINT('',(-1.,-0.2,9.5));
#12137=CARTESIAN_POINT('',(-1.,-0.2,7.5));
#12138=CARTESIAN_POINT('Origin',(-1.,1.8,7.5));
#12139=CARTESIAN_POINT('',(-1.,0.817949192431123,7.5));
#12140=CARTESIAN_POINT('',(-1.,1.8,7.5));
#12141=CARTESIAN_POINT('',(-1.,1.3,7.5));
#12142=CARTESIAN_POINT('',(-1.,1.8,9.5));
#12143=CARTESIAN_POINT('Origin',(0.,0.8,9.5));
#12144=CARTESIAN_POINT('Origin',(0.,0.8,7.5));
#12145=CARTESIAN_POINT('',(-0.505181485540922,1.675,7.5));
#12146=CARTESIAN_POINT('',(-0.505181485540922,1.675,7.5));
#12147=CARTESIAN_POINT('',(0.505181485540923,1.675,7.5));
#12148=CARTESIAN_POINT('',(1.01036297108185,0.8,7.5));
#12149=CARTESIAN_POINT('',(0.505181485540923,1.675,7.5));
#12150=CARTESIAN_POINT('Origin',(0.,0.8,7.5));
#12151=CARTESIAN_POINT('',(1.01036297108185,0.8,7.5));
#12152=CARTESIAN_POINT('',(0.505181485540923,-0.075,7.5));
#12153=CARTESIAN_POINT('',(1.01036297108185,0.8,7.5));
#12154=CARTESIAN_POINT('Origin',(0.,0.8,7.));
#12155=CARTESIAN_POINT('',(0.505181485540923,-0.075,7.));
#12156=CARTESIAN_POINT('',(1.01036297108185,0.8,7.));
#12157=CARTESIAN_POINT('',(0.505181485540923,-0.075,7.));
#12158=CARTESIAN_POINT('',(-0.505181485540923,-0.0749999999999997,7.));
#12159=CARTESIAN_POINT('',(-0.505181485540923,-0.0749999999999997,7.));
#12160=CARTESIAN_POINT('',(-1.01036297108185,0.8,7.));
#12161=CARTESIAN_POINT('',(-1.01036297108185,0.8,7.));
#12162=CARTESIAN_POINT('',(-0.505181485540922,1.675,7.));
#12163=CARTESIAN_POINT('',(-0.505181485540922,1.675,7.));
#12164=CARTESIAN_POINT('',(0.505181485540923,1.675,7.));
#12165=CARTESIAN_POINT('',(0.505181485540923,1.675,7.));
#12166=CARTESIAN_POINT('',(1.01036297108185,0.8,7.));
#12167=CARTESIAN_POINT('',(-0.685,0.8,7.));
#12168=CARTESIAN_POINT('Origin',(0.,0.8,7.));
#12169=CARTESIAN_POINT('Origin',(-0.505181485540923,-0.0749999999999997,
7.));
#12170=CARTESIAN_POINT('',(0.505181485540923,-0.075,7.));
#12171=CARTESIAN_POINT('',(-0.505181485540923,-0.0749999999999997,7.));
#12172=CARTESIAN_POINT('Origin',(-1.01036297108185,0.8,7.));
#12173=CARTESIAN_POINT('',(-1.01036297108185,0.8,7.5));
#12174=CARTESIAN_POINT('',(-1.01036297108185,0.8,7.5));
#12175=CARTESIAN_POINT('',(-1.01036297108185,0.8,7.));
#12176=CARTESIAN_POINT('Origin',(-0.505181485540922,1.675,7.));
#12177=CARTESIAN_POINT('',(-0.505181485540922,1.675,7.5));
#12178=CARTESIAN_POINT('',(-0.505181485540922,1.675,7.));
#12179=CARTESIAN_POINT('Origin',(0.505181485540923,1.675,7.));
#12180=CARTESIAN_POINT('',(0.505181485540923,1.675,7.));
#12181=CARTESIAN_POINT('Origin',(1.01036297108185,0.8,7.));
#12182=CARTESIAN_POINT('',(1.01036297108185,0.8,7.));
#12183=CARTESIAN_POINT('Origin',(0.505181485540923,-0.075,7.));
#12184=CARTESIAN_POINT('Origin',(0.,0.8,7.5));
#12185=CARTESIAN_POINT('Origin',(0.,0.8,5.8));
#12186=CARTESIAN_POINT('',(-0.2,0.8,5.8));
#12187=CARTESIAN_POINT('',(-0.2,0.8,5.8));
#12188=CARTESIAN_POINT('Origin',(0.,0.8,5.8));
#12189=CARTESIAN_POINT('Origin',(0.,0.8,5.8));
#12190=CARTESIAN_POINT('',(-0.685,0.8,5.8));
#12191=CARTESIAN_POINT('',(-0.685,0.8,5.8));
#12192=CARTESIAN_POINT('Origin',(0.,0.8,5.8));
#12193=CARTESIAN_POINT('Origin',(0.,0.8,5.8));
#14300=UNCERTAINTY_MEASURE_WITH_UNIT(LENGTH_MEASURE(0.001),#14393,
'DISTANCE_ACCURACY_VALUE',
'Maximum model space distance between geometric entities at asserted c
onnectivities');
#14344=UNCERTAINTY_MEASURE_WITH_UNIT(LENGTH_MEASURE(0.001),#14393,
'DISTANCE_ACCURACY_VALUE',
'Maximum model space distance between geometric entities at asserted c
onnectivities');
#14348=(
GEOMETRIC_REPRESENTATION_CONTEXT(3)
GLOBAL_UNCERTAINTY_ASSIGNED_CONTEXT((#14300))
GLOBAL_UNIT_ASSIGNED_CONTEXT((#14393,#14395,#14396))
REPRESENTATION_CONTEXT('','3D')
);
#14392=(
GEOMETRIC_REPRESENTATION_CONTEXT(3)
GLOBAL_UNCERTAINTY_ASSIGNED_CONTEXT((#14344))
GLOBAL_UNIT_ASSIGNED_CONTEXT((#14393,#14395,#14396))
REPRESENTATION_CONTEXT('','3D')
);
#14393=(
LENGTH_UNIT()
NAMED_UNIT(*)
SI_UNIT(.CENTI.,.METRE.)
);
#14395=(
NAMED_UNIT(*)
PLANE_ANGLE_UNIT()
SI_UNIT($,.RADIAN.)
);
#14396=(
NAMED_UNIT(*)
SI_UNIT($,.STERADIAN.)
SOLID_ANGLE_UNIT()
);
#14400=SHAPE_DEFINITION_REPRESENTATION(#14447,#14586);
#14447=PRODUCT_DEFINITION_SHAPE('',$,#14634);
#14586=SHAPE_REPRESENTATION('',(#8456),#14348);
#14630=PRODUCT_DEFINITION_CONTEXT('part definition',#14773,'design');
#14634=PRODUCT_DEFINITION('Needle flow-control fitting',
'Needle flow-control fitting',#14681,#14630);
#14681=PRODUCT_DEFINITION_FORMATION('',$,#14778);
#14773=APPLICATION_CONTEXT(
'Core Data for Automotive Mechanical Design Process');
#14774=PRODUCT_CONTEXT('part definition',#14773,'mechanical');
#14778=PRODUCT('Needle flow-control fitting',
'Needle flow-control fitting','Needle flow-control fitting',(#14774));
#14878=COLOUR_RGB('Sky Blue',0.24,0.69,0.87);
#14879=FILL_AREA_STYLE_COLOUR('',#14878);
#14880=FILL_AREA_STYLE('',(#14879));
#14881=SURFACE_STYLE_FILL_AREA(#14880);
#14882=SURFACE_SIDE_STYLE('',(#14881));
#14883=SURFACE_STYLE_USAGE(.BOTH.,#14882);
#14884=PRESENTATION_STYLE_ASSIGNMENT((#14883));
ENDSEC;
END-ISO-10303-21;
